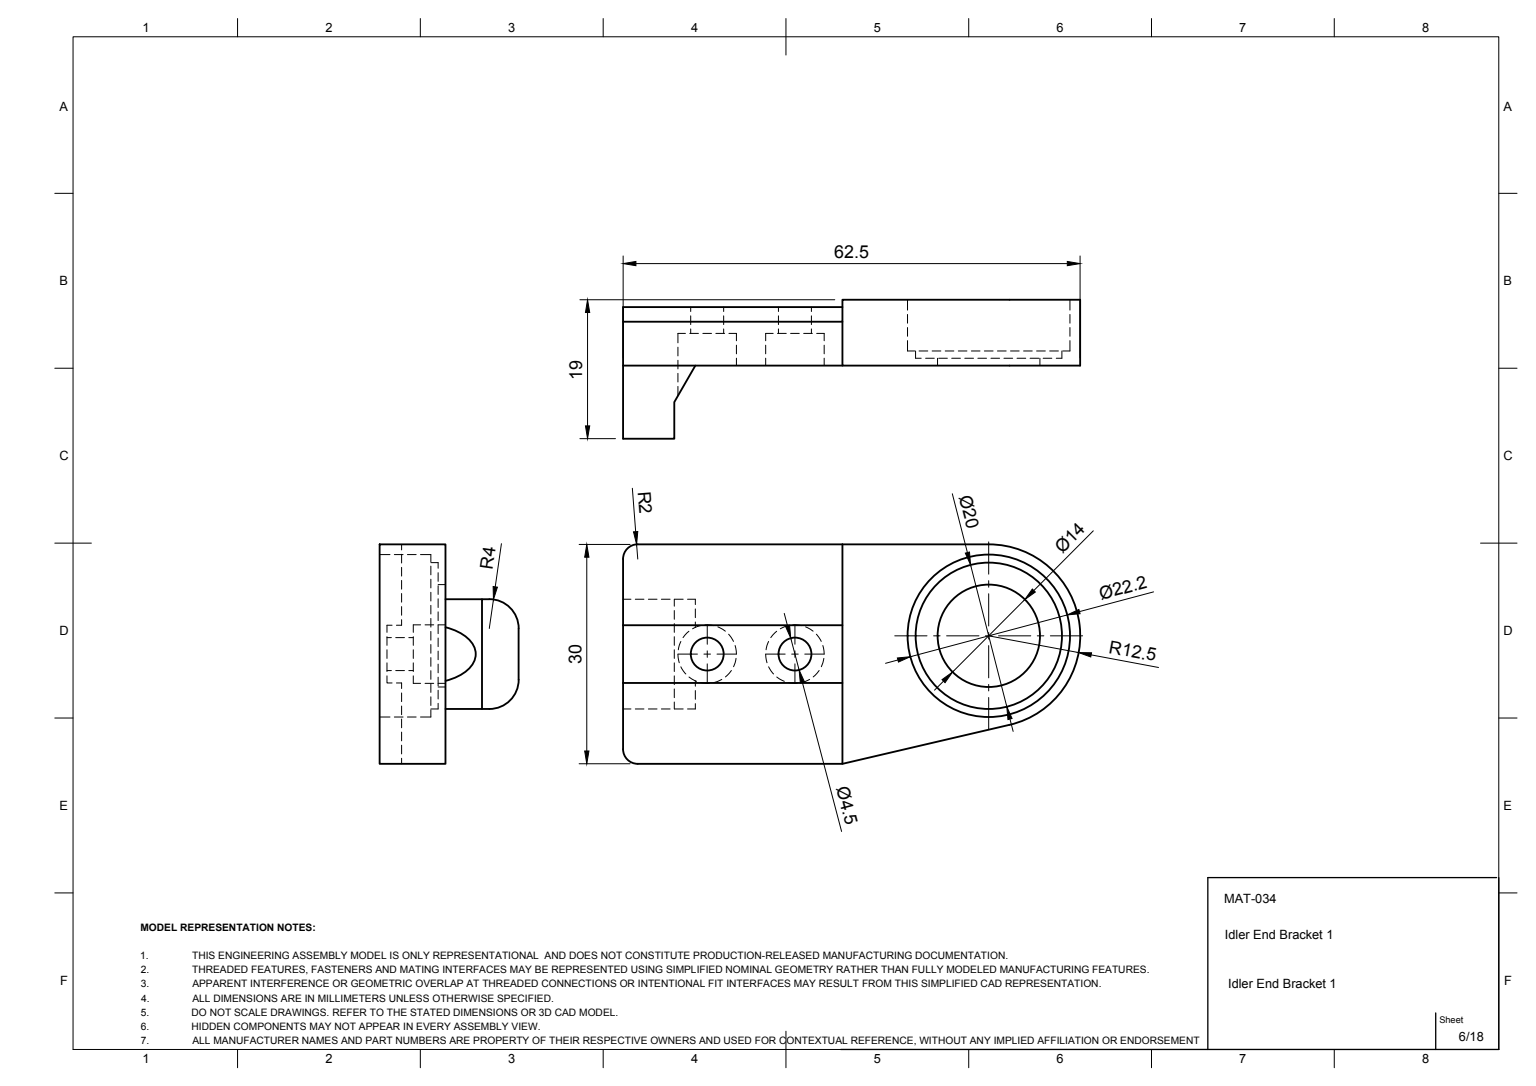
ISO-10303-21;
HEADER;
/* Generated by software containing ST-Developer
 * from STEP Tools, Inc. (www.steptools.com) 
 */

FILE_DESCRIPTION(
/* description */ ('STEP AP214'),
/* implementation_level */ '2;1');

FILE_NAME(
/* name */ 'Idler End Bracket 1.step',
/* time_stamp */ '2026-11-14T09:24:36-08:00',
/* author */ (''),
/* organization */ (''),
/* preprocessor_version */ 'ST-DEVELOPER v20.2',
/* originating_system */ 'Autodesk Translation Framework v15.17.0.0',
/* authorisation */ '');

FILE_SCHEMA (('AUTOMOTIVE_DESIGN { 1 0 10303 214 3 1 1 }'));
ENDSEC;

DATA;
#10=MECHANICAL_DESIGN_GEOMETRIC_PRESENTATION_REPRESENTATION('',(#205),#18867);
#167=ELLIPSE('',#11309,7.99999999999913,3.99999999999963);
#168=ELLIPSE('',#11311,7.99999999999913,3.99999999999963);
#173=SHAPE_REPRESENTATION_RELATIONSHIP('SRR','None',#18937,#189);
#189=ADVANCED_BREP_SHAPE_REPRESENTATION('',(#229),#18853);
#205=STYLED_ITEM('',(#19024),#229);
#229=MANIFOLD_SOLID_BREP('Body1',#10960);
#283=FACE_BOUND('',#1465,.T.);
#284=FACE_BOUND('',#1466,.T.);
#285=FACE_BOUND('',#1468,.T.);
#286=FACE_BOUND('',#1470,.T.);
#287=FACE_BOUND('',#1472,.T.);
#288=FACE_BOUND('',#1476,.T.);
#289=FACE_BOUND('',#1478,.T.);
#290=FACE_BOUND('',#1487,.T.);
#291=FACE_BOUND('',#1488,.T.);
#453=PLANE('',#11330);
#454=PLANE('',#11332);
#455=PLANE('',#11334);
#456=PLANE('',#11335);
#457=PLANE('',#11339);
#458=PLANE('',#11340);
#459=PLANE('',#11343);
#460=PLANE('',#11344);
#461=PLANE('',#11347);
#462=PLANE('',#11348);
#463=PLANE('',#11349);
#464=PLANE('',#11352);
#465=PLANE('',#11353);
#466=PLANE('',#11354);
#467=PLANE('',#11355);
#468=PLANE('',#11358);
#469=PLANE('',#11359);
#470=PLANE('',#11362);
#471=PLANE('',#11363);
#472=PLANE('',#11364);
#473=PLANE('',#11365);
#821=FACE_OUTER_BOUND('',#1449,.T.);
#822=FACE_OUTER_BOUND('',#1450,.T.);
#823=FACE_OUTER_BOUND('',#1451,.T.);
#824=FACE_OUTER_BOUND('',#1452,.T.);
#825=FACE_OUTER_BOUND('',#1453,.T.);
#826=FACE_OUTER_BOUND('',#1454,.T.);
#827=FACE_OUTER_BOUND('',#1455,.T.);
#828=FACE_OUTER_BOUND('',#1456,.T.);
#829=FACE_OUTER_BOUND('',#1457,.T.);
#830=FACE_OUTER_BOUND('',#1458,.T.);
#831=FACE_OUTER_BOUND('',#1459,.T.);
#832=FACE_OUTER_BOUND('',#1460,.T.);
#833=FACE_OUTER_BOUND('',#1461,.T.);
#834=FACE_OUTER_BOUND('',#1462,.T.);
#835=FACE_OUTER_BOUND('',#1463,.T.);
#836=FACE_OUTER_BOUND('',#1464,.T.);
#837=FACE_OUTER_BOUND('',#1467,.T.);
#838=FACE_OUTER_BOUND('',#1469,.T.);
#839=FACE_OUTER_BOUND('',#1471,.T.);
#840=FACE_OUTER_BOUND('',#1473,.T.);
#841=FACE_OUTER_BOUND('',#1474,.T.);
#842=FACE_OUTER_BOUND('',#1475,.T.);
#843=FACE_OUTER_BOUND('',#1477,.T.);
#844=FACE_OUTER_BOUND('',#1479,.T.);
#845=FACE_OUTER_BOUND('',#1480,.T.);
#846=FACE_OUTER_BOUND('',#1481,.T.);
#847=FACE_OUTER_BOUND('',#1482,.T.);
#848=FACE_OUTER_BOUND('',#1483,.T.);
#849=FACE_OUTER_BOUND('',#1484,.T.);
#850=FACE_OUTER_BOUND('',#1485,.T.);
#851=FACE_OUTER_BOUND('',#1486,.T.);
#852=FACE_OUTER_BOUND('',#1489,.T.);
#853=FACE_OUTER_BOUND('',#1490,.T.);
#1449=EDGE_LOOP('',(#7584,#7585,#7586,#7587,#7588,#7589));
#1450=EDGE_LOOP('',(#7590,#7591,#7592,#7593));
#1451=EDGE_LOOP('',(#7594,#7595,#7596,#7597));
#1452=EDGE_LOOP('',(#7598,#7599,#7600,#7601));
#1453=EDGE_LOOP('',(#7602,#7603,#7604,#7605));
#1454=EDGE_LOOP('',(#7606,#7607,#7608,#7609));
#1455=EDGE_LOOP('',(#7610,#7611,#7612,#7613));
#1456=EDGE_LOOP('',(#7614,#7615,#7616,#7617,#7618));
#1457=EDGE_LOOP('',(#7619,#7620,#7621,#7622,#7623));
#1458=EDGE_LOOP('',(#7624,#7625,#7626,#7627,#7628,#7629,#7630,#7631));
#1459=EDGE_LOOP('',(#7632,#7633,#7634,#7635,#7636));
#1460=EDGE_LOOP('',(#7637,#7638,#7639,#7640));
#1461=EDGE_LOOP('',(#7641,#7642,#7643,#7644,#7645,#7646));
#1462=EDGE_LOOP('',(#7647,#7648,#7649,#7650,#7651,#7652,#7653,#7654,#7655,
#7656,#7657,#7658,#7659,#7660));
#1463=EDGE_LOOP('',(#7661,#7662,#7663,#7664));
#1464=EDGE_LOOP('',(#7665,#7666,#7667,#7668,#7669,#7670,#7671,#7672,#7673,
#7674,#7675,#7676,#7677));
#1465=EDGE_LOOP('',(#7678));
#1466=EDGE_LOOP('',(#7679));
#1467=EDGE_LOOP('',(#7680,#7681,#7682,#7683));
#1468=EDGE_LOOP('',(#7684));
#1469=EDGE_LOOP('',(#7685));
#1470=EDGE_LOOP('',(#7686));
#1471=EDGE_LOOP('',(#7687));
#1472=EDGE_LOOP('',(#7688));
#1473=EDGE_LOOP('',(#7689,#7690,#7691,#7692));
#1474=EDGE_LOOP('',(#7693,#7694,#7695,#7696));
#1475=EDGE_LOOP('',(#7697));
#1476=EDGE_LOOP('',(#7698));
#1477=EDGE_LOOP('',(#7699));
#1478=EDGE_LOOP('',(#7700));
#1479=EDGE_LOOP('',(#7701,#7702,#7703,#7704,#7705));
#1480=EDGE_LOOP('',(#7706,#7707,#7708,#7709,#7710,#7711));
#1481=EDGE_LOOP('',(#7712,#7713,#7714,#7715,#7716));
#1482=EDGE_LOOP('',(#7717,#7718,#7719,#7720));
#1483=EDGE_LOOP('',(#7721,#7722,#7723,#7724));
#1484=EDGE_LOOP('',(#7725,#7726,#7727,#7728));
#1485=EDGE_LOOP('',(#7729,#7730,#7731,#7732,#7733,#7734,#7735));
#1486=EDGE_LOOP('',(#7736,#7737,#7738,#7739));
#1487=EDGE_LOOP('',(#7740));
#1488=EDGE_LOOP('',(#7741));
#1489=EDGE_LOOP('',(#7742,#7743,#7744,#7745));
#1490=EDGE_LOOP('',(#7746,#7747,#7748,#7749));
#2237=LINE('',#16105,#3251);
#2238=LINE('',#16115,#3252);
#2239=LINE('',#16121,#3253);
#2240=LINE('',#16127,#3254);
#2241=LINE('',#16133,#3255);
#2242=LINE('',#16139,#3256);
#2243=LINE('',#16145,#3257);
#2244=LINE('',#16150,#3258);
#2245=LINE('',#16152,#3259);
#2246=LINE('',#16154,#3260);
#2247=LINE('',#16157,#3261);
#2248=LINE('',#16161,#3262);
#2249=LINE('',#16163,#3263);
#2250=LINE('',#16167,#3264);
#2251=LINE('',#16168,#3265);
#2252=LINE('',#16171,#3266);
#2253=LINE('',#16173,#3267);
#2254=LINE('',#16174,#3268);
#2255=LINE('',#16176,#3269);
#2256=LINE('',#16178,#3270);
#2257=LINE('',#16179,#3271);
#2258=LINE('',#16182,#3272);
#2259=LINE('',#16184,#3273);
#2260=LINE('',#16186,#3274);
#2261=LINE('',#16187,#3275);
#2262=LINE('',#16193,#3276);
#2263=LINE('',#16195,#3277);
#2264=LINE('',#16197,#3278);
#2265=LINE('',#16198,#3279);
#2266=LINE('',#16201,#3280);
#2267=LINE('',#16203,#3281);
#2268=LINE('',#16205,#3282);
#2269=LINE('',#16209,#3283);
#2270=LINE('',#16213,#3284);
#2271=LINE('',#16215,#3285);
#2272=LINE('',#16216,#3286);
#2273=LINE('',#16218,#3287);
#2274=LINE('',#16220,#3288);
#2275=LINE('',#16221,#3289);
#2276=LINE('',#16224,#3290);
#2277=LINE('',#16225,#3291);
#2278=LINE('',#16228,#3292);
#2279=LINE('',#16232,#3293);
#2280=LINE('',#16233,#3294);
#2281=LINE('',#16234,#3295);
#2282=LINE('',#16245,#3296);
#2283=LINE('',#16246,#3297);
#2284=LINE('',#16247,#3298);
#2285=LINE('',#16252,#3299);
#2286=LINE('',#16256,#3300);
#2287=LINE('',#16257,#3301);
#2288=LINE('',#16259,#3302);
#2289=LINE('',#16260,#3303);
#2290=LINE('',#16262,#3304);
#2291=LINE('',#16263,#3305);
#2292=LINE('',#16268,#3306);
#2293=LINE('',#16269,#3307);
#3251=VECTOR('',#12793,4.);
#3252=VECTOR('',#12804,2.25);
#3253=VECTOR('',#12811,4.);
#3254=VECTOR('',#12818,2.25);
#3255=VECTOR('',#12825,7.00000000000001);
#3256=VECTOR('',#12832,10.);
#3257=VECTOR('',#12839,11.1);
#3258=VECTOR('',#12844,1000.);
#3259=VECTOR('',#12845,1000.);
#3260=VECTOR('',#12846,1000.);
#3261=VECTOR('',#12849,1000.);
#3262=VECTOR('',#12852,1000.);
#3263=VECTOR('',#12853,1000.);
#3264=VECTOR('',#12856,1000.);
#3265=VECTOR('',#12857,1000.);
#3266=VECTOR('',#12860,1000.);
#3267=VECTOR('',#12861,1000.);
#3268=VECTOR('',#12862,1000.);
#3269=VECTOR('',#12863,1000.);
#3270=VECTOR('',#12864,1000.);
#3271=VECTOR('',#12865,1000.);
#3272=VECTOR('',#12868,1000.);
#3273=VECTOR('',#12869,1000.);
#3274=VECTOR('',#12870,1000.);
#3275=VECTOR('',#12871,1000.);
#3276=VECTOR('',#12878,1000.);
#3277=VECTOR('',#12881,1000.);
#3278=VECTOR('',#12882,1000.);
#3279=VECTOR('',#12883,1000.);
#3280=VECTOR('',#12886,1000.);
#3281=VECTOR('',#12887,1000.);
#3282=VECTOR('',#12888,1000.);
#3283=VECTOR('',#12891,1000.);
#3284=VECTOR('',#12894,1000.);
#3285=VECTOR('',#12895,1000.);
#3286=VECTOR('',#12896,1000.);
#3287=VECTOR('',#12897,1000.);
#3288=VECTOR('',#12898,1000.);
#3289=VECTOR('',#12899,1000.);
#3290=VECTOR('',#12902,1000.);
#3291=VECTOR('',#12903,1000.);
#3292=VECTOR('',#12906,1000.);
#3293=VECTOR('',#12911,1000.);
#3294=VECTOR('',#12912,1000.);
#3295=VECTOR('',#12913,1000.);
#3296=VECTOR('',#12930,1000.);
#3297=VECTOR('',#12931,1000.);
#3298=VECTOR('',#12932,1000.);
#3299=VECTOR('',#12937,1000.);
#3300=VECTOR('',#12940,1000.);
#3301=VECTOR('',#12941,1000.);
#3302=VECTOR('',#12944,1000.);
#3303=VECTOR('',#12945,1000.);
#3304=VECTOR('',#12948,1000.);
#3305=VECTOR('',#12949,1000.);
#3306=VECTOR('',#12958,1000.);
#3307=VECTOR('',#12959,1000.);
#4123=CIRCLE('',#11308,4.);
#4124=CIRCLE('',#11310,4.);
#4125=CIRCLE('',#11313,2.25);
#4126=CIRCLE('',#11314,2.25);
#4127=CIRCLE('',#11316,4.);
#4128=CIRCLE('',#11317,4.);
#4129=CIRCLE('',#11319,2.25);
#4130=CIRCLE('',#11320,2.25);
#4131=CIRCLE('',#11322,7.00000000000001);
#4132=CIRCLE('',#11323,7.00000000000001);
#4133=CIRCLE('',#11325,10.);
#4134=CIRCLE('',#11326,10.);
#4135=CIRCLE('',#11328,11.1);
#4136=CIRCLE('',#11329,11.1);
#4137=CIRCLE('',#11331,2.);
#4138=CIRCLE('',#11333,2.);
#4139=CIRCLE('',#11337,12.5);
#4140=CIRCLE('',#11338,12.5);
#4141=CIRCLE('',#11341,4.);
#4142=CIRCLE('',#11342,4.);
#4143=CIRCLE('',#11345,2.);
#4144=CIRCLE('',#11346,2.);
#4145=CIRCLE('',#11356,4.);
#4146=CIRCLE('',#11357,4.);
#4732=VERTEX_POINT('',#16102);
#4733=VERTEX_POINT('',#16104);
#4734=VERTEX_POINT('',#16106);
#4735=VERTEX_POINT('',#16108);
#4736=VERTEX_POINT('',#16112);
#4737=VERTEX_POINT('',#16114);
#4738=VERTEX_POINT('',#16118);
#4739=VERTEX_POINT('',#16120);
#4740=VERTEX_POINT('',#16124);
#4741=VERTEX_POINT('',#16126);
#4742=VERTEX_POINT('',#16130);
#4743=VERTEX_POINT('',#16132);
#4744=VERTEX_POINT('',#16136);
#4745=VERTEX_POINT('',#16138);
#4746=VERTEX_POINT('',#16142);
#4747=VERTEX_POINT('',#16144);
#4748=VERTEX_POINT('',#16148);
#4749=VERTEX_POINT('',#16149);
#4750=VERTEX_POINT('',#16151);
#4751=VERTEX_POINT('',#16153);
#4752=VERTEX_POINT('',#16155);
#4753=VERTEX_POINT('',#16159);
#4754=VERTEX_POINT('',#16160);
#4755=VERTEX_POINT('',#16162);
#4756=VERTEX_POINT('',#16164);
#4757=VERTEX_POINT('',#16166);
#4758=VERTEX_POINT('',#16170);
#4759=VERTEX_POINT('',#16172);
#4760=VERTEX_POINT('',#16175);
#4761=VERTEX_POINT('',#16177);
#4762=VERTEX_POINT('',#16181);
#4763=VERTEX_POINT('',#16183);
#4764=VERTEX_POINT('',#16185);
#4765=VERTEX_POINT('',#16189);
#4766=VERTEX_POINT('',#16191);
#4767=VERTEX_POINT('',#16196);
#4768=VERTEX_POINT('',#16200);
#4769=VERTEX_POINT('',#16202);
#4770=VERTEX_POINT('',#16204);
#4771=VERTEX_POINT('',#16206);
#4772=VERTEX_POINT('',#16208);
#4773=VERTEX_POINT('',#16210);
#4774=VERTEX_POINT('',#16212);
#4775=VERTEX_POINT('',#16214);
#4776=VERTEX_POINT('',#16217);
#4777=VERTEX_POINT('',#16219);
#4778=VERTEX_POINT('',#16223);
#4779=VERTEX_POINT('',#16227);
#4780=VERTEX_POINT('',#16231);
#4781=VERTEX_POINT('',#16243);
#4782=VERTEX_POINT('',#16244);
#4783=VERTEX_POINT('',#16249);
#4784=VERTEX_POINT('',#16251);
#4785=VERTEX_POINT('',#16253);
#4786=VERTEX_POINT('',#16255);
#5825=EDGE_CURVE('',#4732,#4732,#4123,.T.);
#5826=EDGE_CURVE('',#4732,#4733,#2237,.T.);
#5827=EDGE_CURVE('',#4734,#4733,#167,.T.);
#5828=EDGE_CURVE('',#4735,#4734,#4124,.T.);
#5829=EDGE_CURVE('',#4733,#4735,#168,.T.);
#5830=EDGE_CURVE('',#4736,#4736,#4125,.T.);
#5831=EDGE_CURVE('',#4736,#4737,#2238,.T.);
#5832=EDGE_CURVE('',#4737,#4737,#4126,.T.);
#5833=EDGE_CURVE('',#4738,#4738,#4127,.T.);
#5834=EDGE_CURVE('',#4738,#4739,#2239,.T.);
#5835=EDGE_CURVE('',#4739,#4739,#4128,.T.);
#5836=EDGE_CURVE('',#4740,#4740,#4129,.T.);
#5837=EDGE_CURVE('',#4740,#4741,#2240,.T.);
#5838=EDGE_CURVE('',#4741,#4741,#4130,.T.);
#5839=EDGE_CURVE('',#4742,#4742,#4131,.T.);
#5840=EDGE_CURVE('',#4742,#4743,#2241,.T.);
#5841=EDGE_CURVE('',#4743,#4743,#4132,.T.);
#5842=EDGE_CURVE('',#4744,#4744,#4133,.T.);
#5843=EDGE_CURVE('',#4744,#4745,#2242,.T.);
#5844=EDGE_CURVE('',#4745,#4745,#4134,.T.);
#5845=EDGE_CURVE('',#4746,#4746,#4135,.T.);
#5846=EDGE_CURVE('',#4746,#4747,#2243,.T.);
#5847=EDGE_CURVE('',#4747,#4747,#4136,.T.);
#5848=EDGE_CURVE('',#4748,#4749,#2244,.T.);
#5849=EDGE_CURVE('',#4749,#4750,#2245,.T.);
#5850=EDGE_CURVE('',#4751,#4750,#2246,.T.);
#5851=EDGE_CURVE('',#4752,#4751,#4137,.T.);
#5852=EDGE_CURVE('',#4748,#4752,#2247,.T.);
#5853=EDGE_CURVE('',#4753,#4754,#2248,.T.);
#5854=EDGE_CURVE('',#4755,#4754,#2249,.T.);
#5855=EDGE_CURVE('',#4756,#4755,#4138,.T.);
#5856=EDGE_CURVE('',#4756,#4757,#2250,.T.);
#5857=EDGE_CURVE('',#4757,#4753,#2251,.T.);
#5858=EDGE_CURVE('',#4758,#4749,#2252,.T.);
#5859=EDGE_CURVE('',#4758,#4759,#2253,.T.);
#5860=EDGE_CURVE('',#4759,#4753,#2254,.T.);
#5861=EDGE_CURVE('',#4757,#4760,#2255,.T.);
#5862=EDGE_CURVE('',#4760,#4761,#2256,.T.);
#5863=EDGE_CURVE('',#4750,#4761,#2257,.T.);
#5864=EDGE_CURVE('',#4762,#4760,#2258,.T.);
#5865=EDGE_CURVE('',#4763,#4757,#2259,.T.);
#5866=EDGE_CURVE('',#4764,#4763,#2260,.T.);
#5867=EDGE_CURVE('',#4764,#4762,#2261,.T.);
#5868=EDGE_CURVE('',#4762,#4765,#4139,.T.);
#5869=EDGE_CURVE('',#4764,#4766,#4140,.T.);
#5870=EDGE_CURVE('',#4766,#4765,#2262,.T.);
#5871=EDGE_CURVE('',#4761,#4765,#2263,.T.);
#5872=EDGE_CURVE('',#4767,#4766,#2264,.T.);
#5873=EDGE_CURVE('',#4751,#4767,#2265,.T.);
#5874=EDGE_CURVE('',#4768,#4752,#2266,.T.);
#5875=EDGE_CURVE('',#4768,#4769,#2267,.T.);
#5876=EDGE_CURVE('',#4770,#4769,#2268,.T.);
#5877=EDGE_CURVE('',#4771,#4770,#4141,.T.);
#5878=EDGE_CURVE('',#4771,#4772,#2269,.T.);
#5879=EDGE_CURVE('',#4773,#4772,#4142,.T.);
#5880=EDGE_CURVE('',#4773,#4774,#2270,.T.);
#5881=EDGE_CURVE('',#4774,#4775,#2271,.T.);
#5882=EDGE_CURVE('',#4755,#4775,#2272,.T.);
#5883=EDGE_CURVE('',#4776,#4754,#2273,.T.);
#5884=EDGE_CURVE('',#4776,#4777,#2274,.T.);
#5885=EDGE_CURVE('',#4777,#4748,#2275,.T.);
#5886=EDGE_CURVE('',#4778,#4756,#2276,.T.);
#5887=EDGE_CURVE('',#4778,#4763,#2277,.T.);
#5888=EDGE_CURVE('',#4779,#4769,#2278,.T.);
#5889=EDGE_CURVE('',#4767,#4768,#4143,.T.);
#5890=EDGE_CURVE('',#4775,#4778,#4144,.T.);
#5891=EDGE_CURVE('',#4774,#4780,#2279,.T.);
#5892=EDGE_CURVE('',#4735,#4780,#2280,.T.);
#5893=EDGE_CURVE('',#4779,#4734,#2281,.T.);
#5894=EDGE_CURVE('',#4781,#4782,#2282,.T.);
#5895=EDGE_CURVE('',#4780,#4782,#2283,.T.);
#5896=EDGE_CURVE('',#4781,#4773,#2284,.T.);
#5897=EDGE_CURVE('',#4783,#4781,#4145,.T.);
#5898=EDGE_CURVE('',#4783,#4784,#2285,.T.);
#5899=EDGE_CURVE('',#4785,#4784,#4146,.T.);
#5900=EDGE_CURVE('',#4785,#4786,#2286,.T.);
#5901=EDGE_CURVE('',#4782,#4786,#2287,.T.);
#5902=EDGE_CURVE('',#4786,#4779,#2288,.T.);
#5903=EDGE_CURVE('',#4770,#4785,#2289,.T.);
#5904=EDGE_CURVE('',#4772,#4783,#2290,.T.);
#5905=EDGE_CURVE('',#4784,#4771,#2291,.T.);
#5906=EDGE_CURVE('',#4759,#4776,#2292,.T.);
#5907=EDGE_CURVE('',#4777,#4758,#2293,.T.);
#7584=ORIENTED_EDGE('',*,*,#5825,.T.);
#7585=ORIENTED_EDGE('',*,*,#5826,.T.);
#7586=ORIENTED_EDGE('',*,*,#5827,.F.);
#7587=ORIENTED_EDGE('',*,*,#5828,.F.);
#7588=ORIENTED_EDGE('',*,*,#5829,.F.);
#7589=ORIENTED_EDGE('',*,*,#5826,.F.);
#7590=ORIENTED_EDGE('',*,*,#5830,.F.);
#7591=ORIENTED_EDGE('',*,*,#5831,.T.);
#7592=ORIENTED_EDGE('',*,*,#5832,.F.);
#7593=ORIENTED_EDGE('',*,*,#5831,.F.);
#7594=ORIENTED_EDGE('',*,*,#5833,.T.);
#7595=ORIENTED_EDGE('',*,*,#5834,.T.);
#7596=ORIENTED_EDGE('',*,*,#5835,.F.);
#7597=ORIENTED_EDGE('',*,*,#5834,.F.);
#7598=ORIENTED_EDGE('',*,*,#5836,.F.);
#7599=ORIENTED_EDGE('',*,*,#5837,.T.);
#7600=ORIENTED_EDGE('',*,*,#5838,.F.);
#7601=ORIENTED_EDGE('',*,*,#5837,.F.);
#7602=ORIENTED_EDGE('',*,*,#5839,.T.);
#7603=ORIENTED_EDGE('',*,*,#5840,.T.);
#7604=ORIENTED_EDGE('',*,*,#5841,.F.);
#7605=ORIENTED_EDGE('',*,*,#5840,.F.);
#7606=ORIENTED_EDGE('',*,*,#5842,.T.);
#7607=ORIENTED_EDGE('',*,*,#5843,.T.);
#7608=ORIENTED_EDGE('',*,*,#5844,.F.);
#7609=ORIENTED_EDGE('',*,*,#5843,.F.);
#7610=ORIENTED_EDGE('',*,*,#5845,.T.);
#7611=ORIENTED_EDGE('',*,*,#5846,.T.);
#7612=ORIENTED_EDGE('',*,*,#5847,.F.);
#7613=ORIENTED_EDGE('',*,*,#5846,.F.);
#7614=ORIENTED_EDGE('',*,*,#5848,.T.);
#7615=ORIENTED_EDGE('',*,*,#5849,.T.);
#7616=ORIENTED_EDGE('',*,*,#5850,.F.);
#7617=ORIENTED_EDGE('',*,*,#5851,.F.);
#7618=ORIENTED_EDGE('',*,*,#5852,.F.);
#7619=ORIENTED_EDGE('',*,*,#5853,.T.);
#7620=ORIENTED_EDGE('',*,*,#5854,.F.);
#7621=ORIENTED_EDGE('',*,*,#5855,.F.);
#7622=ORIENTED_EDGE('',*,*,#5856,.T.);
#7623=ORIENTED_EDGE('',*,*,#5857,.T.);
#7624=ORIENTED_EDGE('',*,*,#5858,.F.);
#7625=ORIENTED_EDGE('',*,*,#5859,.T.);
#7626=ORIENTED_EDGE('',*,*,#5860,.T.);
#7627=ORIENTED_EDGE('',*,*,#5857,.F.);
#7628=ORIENTED_EDGE('',*,*,#5861,.T.);
#7629=ORIENTED_EDGE('',*,*,#5862,.T.);
#7630=ORIENTED_EDGE('',*,*,#5863,.F.);
#7631=ORIENTED_EDGE('',*,*,#5849,.F.);
#7632=ORIENTED_EDGE('',*,*,#5864,.T.);
#7633=ORIENTED_EDGE('',*,*,#5861,.F.);
#7634=ORIENTED_EDGE('',*,*,#5865,.F.);
#7635=ORIENTED_EDGE('',*,*,#5866,.F.);
#7636=ORIENTED_EDGE('',*,*,#5867,.T.);
#7637=ORIENTED_EDGE('',*,*,#5868,.F.);
#7638=ORIENTED_EDGE('',*,*,#5867,.F.);
#7639=ORIENTED_EDGE('',*,*,#5869,.T.);
#7640=ORIENTED_EDGE('',*,*,#5870,.T.);
#7641=ORIENTED_EDGE('',*,*,#5863,.T.);
#7642=ORIENTED_EDGE('',*,*,#5871,.T.);
#7643=ORIENTED_EDGE('',*,*,#5870,.F.);
#7644=ORIENTED_EDGE('',*,*,#5872,.F.);
#7645=ORIENTED_EDGE('',*,*,#5873,.F.);
#7646=ORIENTED_EDGE('',*,*,#5850,.T.);
#7647=ORIENTED_EDGE('',*,*,#5874,.F.);
#7648=ORIENTED_EDGE('',*,*,#5875,.T.);
#7649=ORIENTED_EDGE('',*,*,#5876,.F.);
#7650=ORIENTED_EDGE('',*,*,#5877,.F.);
#7651=ORIENTED_EDGE('',*,*,#5878,.T.);
#7652=ORIENTED_EDGE('',*,*,#5879,.F.);
#7653=ORIENTED_EDGE('',*,*,#5880,.T.);
#7654=ORIENTED_EDGE('',*,*,#5881,.T.);
#7655=ORIENTED_EDGE('',*,*,#5882,.F.);
#7656=ORIENTED_EDGE('',*,*,#5854,.T.);
#7657=ORIENTED_EDGE('',*,*,#5883,.F.);
#7658=ORIENTED_EDGE('',*,*,#5884,.T.);
#7659=ORIENTED_EDGE('',*,*,#5885,.T.);
#7660=ORIENTED_EDGE('',*,*,#5852,.T.);
#7661=ORIENTED_EDGE('',*,*,#5886,.F.);
#7662=ORIENTED_EDGE('',*,*,#5887,.T.);
#7663=ORIENTED_EDGE('',*,*,#5865,.T.);
#7664=ORIENTED_EDGE('',*,*,#5856,.F.);
#7665=ORIENTED_EDGE('',*,*,#5888,.T.);
#7666=ORIENTED_EDGE('',*,*,#5875,.F.);
#7667=ORIENTED_EDGE('',*,*,#5889,.F.);
#7668=ORIENTED_EDGE('',*,*,#5872,.T.);
#7669=ORIENTED_EDGE('',*,*,#5869,.F.);
#7670=ORIENTED_EDGE('',*,*,#5866,.T.);
#7671=ORIENTED_EDGE('',*,*,#5887,.F.);
#7672=ORIENTED_EDGE('',*,*,#5890,.F.);
#7673=ORIENTED_EDGE('',*,*,#5881,.F.);
#7674=ORIENTED_EDGE('',*,*,#5891,.T.);
#7675=ORIENTED_EDGE('',*,*,#5892,.F.);
#7676=ORIENTED_EDGE('',*,*,#5828,.T.);
#7677=ORIENTED_EDGE('',*,*,#5893,.F.);
#7678=ORIENTED_EDGE('',*,*,#5835,.T.);
#7679=ORIENTED_EDGE('',*,*,#5839,.F.);
#7680=ORIENTED_EDGE('',*,*,#5864,.F.);
#7681=ORIENTED_EDGE('',*,*,#5868,.T.);
#7682=ORIENTED_EDGE('',*,*,#5871,.F.);
#7683=ORIENTED_EDGE('',*,*,#5862,.F.);
#7684=ORIENTED_EDGE('',*,*,#5847,.T.);
#7685=ORIENTED_EDGE('',*,*,#5845,.F.);
#7686=ORIENTED_EDGE('',*,*,#5844,.T.);
#7687=ORIENTED_EDGE('',*,*,#5842,.F.);
#7688=ORIENTED_EDGE('',*,*,#5841,.T.);
#7689=ORIENTED_EDGE('',*,*,#5855,.T.);
#7690=ORIENTED_EDGE('',*,*,#5882,.T.);
#7691=ORIENTED_EDGE('',*,*,#5890,.T.);
#7692=ORIENTED_EDGE('',*,*,#5886,.T.);
#7693=ORIENTED_EDGE('',*,*,#5851,.T.);
#7694=ORIENTED_EDGE('',*,*,#5873,.T.);
#7695=ORIENTED_EDGE('',*,*,#5889,.T.);
#7696=ORIENTED_EDGE('',*,*,#5874,.T.);
#7697=ORIENTED_EDGE('',*,*,#5833,.F.);
#7698=ORIENTED_EDGE('',*,*,#5838,.T.);
#7699=ORIENTED_EDGE('',*,*,#5825,.F.);
#7700=ORIENTED_EDGE('',*,*,#5832,.T.);
#7701=ORIENTED_EDGE('',*,*,#5894,.T.);
#7702=ORIENTED_EDGE('',*,*,#5895,.F.);
#7703=ORIENTED_EDGE('',*,*,#5891,.F.);
#7704=ORIENTED_EDGE('',*,*,#5880,.F.);
#7705=ORIENTED_EDGE('',*,*,#5896,.F.);
#7706=ORIENTED_EDGE('',*,*,#5894,.F.);
#7707=ORIENTED_EDGE('',*,*,#5897,.F.);
#7708=ORIENTED_EDGE('',*,*,#5898,.T.);
#7709=ORIENTED_EDGE('',*,*,#5899,.F.);
#7710=ORIENTED_EDGE('',*,*,#5900,.T.);
#7711=ORIENTED_EDGE('',*,*,#5901,.F.);
#7712=ORIENTED_EDGE('',*,*,#5876,.T.);
#7713=ORIENTED_EDGE('',*,*,#5888,.F.);
#7714=ORIENTED_EDGE('',*,*,#5902,.F.);
#7715=ORIENTED_EDGE('',*,*,#5900,.F.);
#7716=ORIENTED_EDGE('',*,*,#5903,.F.);
#7717=ORIENTED_EDGE('',*,*,#5898,.F.);
#7718=ORIENTED_EDGE('',*,*,#5904,.F.);
#7719=ORIENTED_EDGE('',*,*,#5878,.F.);
#7720=ORIENTED_EDGE('',*,*,#5905,.F.);
#7721=ORIENTED_EDGE('',*,*,#5899,.T.);
#7722=ORIENTED_EDGE('',*,*,#5905,.T.);
#7723=ORIENTED_EDGE('',*,*,#5877,.T.);
#7724=ORIENTED_EDGE('',*,*,#5903,.T.);
#7725=ORIENTED_EDGE('',*,*,#5879,.T.);
#7726=ORIENTED_EDGE('',*,*,#5904,.T.);
#7727=ORIENTED_EDGE('',*,*,#5897,.T.);
#7728=ORIENTED_EDGE('',*,*,#5896,.T.);
#7729=ORIENTED_EDGE('',*,*,#5827,.T.);
#7730=ORIENTED_EDGE('',*,*,#5829,.T.);
#7731=ORIENTED_EDGE('',*,*,#5892,.T.);
#7732=ORIENTED_EDGE('',*,*,#5895,.T.);
#7733=ORIENTED_EDGE('',*,*,#5901,.T.);
#7734=ORIENTED_EDGE('',*,*,#5902,.T.);
#7735=ORIENTED_EDGE('',*,*,#5893,.T.);
#7736=ORIENTED_EDGE('',*,*,#5884,.F.);
#7737=ORIENTED_EDGE('',*,*,#5906,.F.);
#7738=ORIENTED_EDGE('',*,*,#5859,.F.);
#7739=ORIENTED_EDGE('',*,*,#5907,.F.);
#7740=ORIENTED_EDGE('',*,*,#5830,.T.);
#7741=ORIENTED_EDGE('',*,*,#5836,.T.);
#7742=ORIENTED_EDGE('',*,*,#5848,.F.);
#7743=ORIENTED_EDGE('',*,*,#5885,.F.);
#7744=ORIENTED_EDGE('',*,*,#5907,.T.);
#7745=ORIENTED_EDGE('',*,*,#5858,.T.);
#7746=ORIENTED_EDGE('',*,*,#5853,.F.);
#7747=ORIENTED_EDGE('',*,*,#5860,.F.);
#7748=ORIENTED_EDGE('',*,*,#5906,.T.);
#7749=ORIENTED_EDGE('',*,*,#5883,.T.);
#10174=CYLINDRICAL_SURFACE('',#11307,4.);
#10175=CYLINDRICAL_SURFACE('',#11312,2.25);
#10176=CYLINDRICAL_SURFACE('',#11315,4.);
#10177=CYLINDRICAL_SURFACE('',#11318,2.25);
#10178=CYLINDRICAL_SURFACE('',#11321,7.00000000000001);
#10179=CYLINDRICAL_SURFACE('',#11324,10.);
#10180=CYLINDRICAL_SURFACE('',#11327,11.1);
#10181=CYLINDRICAL_SURFACE('',#11336,12.5);
#10182=CYLINDRICAL_SURFACE('',#11350,2.);
#10183=CYLINDRICAL_SURFACE('',#11351,2.);
#10184=CYLINDRICAL_SURFACE('',#11360,4.);
#10185=CYLINDRICAL_SURFACE('',#11361,4.);
#10458=ADVANCED_FACE('',(#821),#10174,.F.);
#10459=ADVANCED_FACE('',(#822),#10175,.F.);
#10460=ADVANCED_FACE('',(#823),#10176,.F.);
#10461=ADVANCED_FACE('',(#824),#10177,.F.);
#10462=ADVANCED_FACE('',(#825),#10178,.F.);
#10463=ADVANCED_FACE('',(#826),#10179,.F.);
#10464=ADVANCED_FACE('',(#827),#10180,.F.);
#10465=ADVANCED_FACE('',(#828),#453,.F.);
#10466=ADVANCED_FACE('',(#829),#454,.F.);
#10467=ADVANCED_FACE('',(#830),#455,.F.);
#10468=ADVANCED_FACE('',(#831),#456,.T.);
#10469=ADVANCED_FACE('',(#832),#10181,.T.);
#10470=ADVANCED_FACE('',(#833),#457,.T.);
#10471=ADVANCED_FACE('',(#834),#458,.F.);
#10472=ADVANCED_FACE('',(#835),#459,.F.);
#10473=ADVANCED_FACE('',(#836,#283,#284),#460,.T.);
#10474=ADVANCED_FACE('',(#837,#285),#461,.F.);
#10475=ADVANCED_FACE('',(#838,#286),#462,.T.);
#10476=ADVANCED_FACE('',(#839,#287),#463,.T.);
#10477=ADVANCED_FACE('',(#840),#10182,.T.);
#10478=ADVANCED_FACE('',(#841),#10183,.T.);
#10479=ADVANCED_FACE('',(#842,#288),#464,.F.);
#10480=ADVANCED_FACE('',(#843,#289),#465,.F.);
#10481=ADVANCED_FACE('',(#844),#466,.F.);
#10482=ADVANCED_FACE('',(#845),#467,.F.);
#10483=ADVANCED_FACE('',(#846),#468,.F.);
#10484=ADVANCED_FACE('',(#847),#469,.T.);
#10485=ADVANCED_FACE('',(#848),#10184,.T.);
#10486=ADVANCED_FACE('',(#849),#10185,.T.);
#10487=ADVANCED_FACE('',(#850),#470,.F.);
#10488=ADVANCED_FACE('',(#851,#290,#291),#471,.F.);
#10489=ADVANCED_FACE('',(#852),#472,.F.);
#10490=ADVANCED_FACE('',(#853),#473,.F.);
#10960=CLOSED_SHELL('',(#10458,#10459,#10460,#10461,#10462,#10463,#10464,
#10465,#10466,#10467,#10468,#10469,#10470,#10471,#10472,#10473,#10474,#10475,
#10476,#10477,#10478,#10479,#10480,#10481,#10482,#10483,#10484,#10485,#10486,
#10487,#10488,#10489,#10490));
#11306=AXIS2_PLACEMENT_3D('',#16100,#12787,#12788);
#11307=AXIS2_PLACEMENT_3D('',#16101,#12789,#12790);
#11308=AXIS2_PLACEMENT_3D('',#16103,#12791,#12792);
#11309=AXIS2_PLACEMENT_3D('',#16107,#12794,#12795);
#11310=AXIS2_PLACEMENT_3D('',#16109,#12796,#12797);
#11311=AXIS2_PLACEMENT_3D('',#16110,#12798,#12799);
#11312=AXIS2_PLACEMENT_3D('',#16111,#12800,#12801);
#11313=AXIS2_PLACEMENT_3D('',#16113,#12802,#12803);
#11314=AXIS2_PLACEMENT_3D('',#16116,#12805,#12806);
#11315=AXIS2_PLACEMENT_3D('',#16117,#12807,#12808);
#11316=AXIS2_PLACEMENT_3D('',#16119,#12809,#12810);
#11317=AXIS2_PLACEMENT_3D('',#16122,#12812,#12813);
#11318=AXIS2_PLACEMENT_3D('',#16123,#12814,#12815);
#11319=AXIS2_PLACEMENT_3D('',#16125,#12816,#12817);
#11320=AXIS2_PLACEMENT_3D('',#16128,#12819,#12820);
#11321=AXIS2_PLACEMENT_3D('',#16129,#12821,#12822);
#11322=AXIS2_PLACEMENT_3D('',#16131,#12823,#12824);
#11323=AXIS2_PLACEMENT_3D('',#16134,#12826,#12827);
#11324=AXIS2_PLACEMENT_3D('',#16135,#12828,#12829);
#11325=AXIS2_PLACEMENT_3D('',#16137,#12830,#12831);
#11326=AXIS2_PLACEMENT_3D('',#16140,#12833,#12834);
#11327=AXIS2_PLACEMENT_3D('',#16141,#12835,#12836);
#11328=AXIS2_PLACEMENT_3D('',#16143,#12837,#12838);
#11329=AXIS2_PLACEMENT_3D('',#16146,#12840,#12841);
#11330=AXIS2_PLACEMENT_3D('',#16147,#12842,#12843);
#11331=AXIS2_PLACEMENT_3D('',#16156,#12847,#12848);
#11332=AXIS2_PLACEMENT_3D('',#16158,#12850,#12851);
#11333=AXIS2_PLACEMENT_3D('',#16165,#12854,#12855);
#11334=AXIS2_PLACEMENT_3D('',#16169,#12858,#12859);
#11335=AXIS2_PLACEMENT_3D('',#16180,#12866,#12867);
#11336=AXIS2_PLACEMENT_3D('',#16188,#12872,#12873);
#11337=AXIS2_PLACEMENT_3D('',#16190,#12874,#12875);
#11338=AXIS2_PLACEMENT_3D('',#16192,#12876,#12877);
#11339=AXIS2_PLACEMENT_3D('',#16194,#12879,#12880);
#11340=AXIS2_PLACEMENT_3D('',#16199,#12884,#12885);
#11341=AXIS2_PLACEMENT_3D('',#16207,#12889,#12890);
#11342=AXIS2_PLACEMENT_3D('',#16211,#12892,#12893);
#11343=AXIS2_PLACEMENT_3D('',#16222,#12900,#12901);
#11344=AXIS2_PLACEMENT_3D('',#16226,#12904,#12905);
#11345=AXIS2_PLACEMENT_3D('',#16229,#12907,#12908);
#11346=AXIS2_PLACEMENT_3D('',#16230,#12909,#12910);
#11347=AXIS2_PLACEMENT_3D('',#16235,#12914,#12915);
#11348=AXIS2_PLACEMENT_3D('',#16236,#12916,#12917);
#11349=AXIS2_PLACEMENT_3D('',#16237,#12918,#12919);
#11350=AXIS2_PLACEMENT_3D('',#16238,#12920,#12921);
#11351=AXIS2_PLACEMENT_3D('',#16239,#12922,#12923);
#11352=AXIS2_PLACEMENT_3D('',#16240,#12924,#12925);
#11353=AXIS2_PLACEMENT_3D('',#16241,#12926,#12927);
#11354=AXIS2_PLACEMENT_3D('',#16242,#12928,#12929);
#11355=AXIS2_PLACEMENT_3D('',#16248,#12933,#12934);
#11356=AXIS2_PLACEMENT_3D('',#16250,#12935,#12936);
#11357=AXIS2_PLACEMENT_3D('',#16254,#12938,#12939);
#11358=AXIS2_PLACEMENT_3D('',#16258,#12942,#12943);
#11359=AXIS2_PLACEMENT_3D('',#16261,#12946,#12947);
#11360=AXIS2_PLACEMENT_3D('',#16264,#12950,#12951);
#11361=AXIS2_PLACEMENT_3D('',#16265,#12952,#12953);
#11362=AXIS2_PLACEMENT_3D('',#16266,#12954,#12955);
#11363=AXIS2_PLACEMENT_3D('',#16267,#12956,#12957);
#11364=AXIS2_PLACEMENT_3D('',#16270,#12960,#12961);
#11365=AXIS2_PLACEMENT_3D('',#16271,#12962,#12963);
#12787=DIRECTION('axis',(0.,0.,1.));
#12788=DIRECTION('refdir',(1.,0.,0.));
#12789=DIRECTION('center_axis',(0.,0.,-1.));
#12790=DIRECTION('ref_axis',(1.,0.,0.));
#12791=DIRECTION('center_axis',(0.,0.,1.));
#12792=DIRECTION('ref_axis',(1.,0.,0.));
#12793=DIRECTION('',(0.,0.,-1.));
#12794=DIRECTION('center_axis',(-0.866025403784435,4.41270772476077E-16,
0.500000000000006));
#12795=DIRECTION('ref_axis',(0.500000000000006,5.55042661661472E-14,0.866025403784435));
#12796=DIRECTION('center_axis',(0.,0.,1.));
#12797=DIRECTION('ref_axis',(1.,0.,0.));
#12798=DIRECTION('center_axis',(-0.866025403784435,4.41270772476077E-16,
0.500000000000006));
#12799=DIRECTION('ref_axis',(0.500000000000006,5.55042661661472E-14,0.866025403784435));
#12800=DIRECTION('center_axis',(0.,0.,-1.));
#12801=DIRECTION('ref_axis',(1.,0.,0.));
#12802=DIRECTION('center_axis',(0.,0.,-1.));
#12803=DIRECTION('ref_axis',(-1.,0.,0.));
#12804=DIRECTION('',(0.,0.,-1.));
#12805=DIRECTION('center_axis',(0.,0.,1.));
#12806=DIRECTION('ref_axis',(1.,0.,0.));
#12807=DIRECTION('center_axis',(0.,0.,-1.));
#12808=DIRECTION('ref_axis',(1.,0.,0.));
#12809=DIRECTION('center_axis',(0.,0.,1.));
#12810=DIRECTION('ref_axis',(1.,0.,0.));
#12811=DIRECTION('',(0.,0.,-1.));
#12812=DIRECTION('center_axis',(0.,0.,1.));
#12813=DIRECTION('ref_axis',(1.,0.,0.));
#12814=DIRECTION('center_axis',(0.,0.,-1.));
#12815=DIRECTION('ref_axis',(1.,0.,0.));
#12816=DIRECTION('center_axis',(0.,0.,-1.));
#12817=DIRECTION('ref_axis',(-1.,0.,0.));
#12818=DIRECTION('',(0.,0.,-1.));
#12819=DIRECTION('center_axis',(0.,0.,1.));
#12820=DIRECTION('ref_axis',(1.,0.,0.));
#12821=DIRECTION('center_axis',(0.,0.,1.));
#12822=DIRECTION('ref_axis',(-1.,0.,0.));
#12823=DIRECTION('center_axis',(0.,0.,-1.));
#12824=DIRECTION('ref_axis',(-1.,0.,0.));
#12825=DIRECTION('',(0.,0.,1.));
#12826=DIRECTION('center_axis',(0.,0.,-1.));
#12827=DIRECTION('ref_axis',(-1.,0.,0.));
#12828=DIRECTION('center_axis',(0.,0.,1.));
#12829=DIRECTION('ref_axis',(-1.,0.,0.));
#12830=DIRECTION('center_axis',(0.,0.,-1.));
#12831=DIRECTION('ref_axis',(-1.,0.,0.));
#12832=DIRECTION('',(0.,0.,1.));
#12833=DIRECTION('center_axis',(0.,0.,-1.));
#12834=DIRECTION('ref_axis',(-1.,0.,0.));
#12835=DIRECTION('center_axis',(0.,0.,1.));
#12836=DIRECTION('ref_axis',(-1.,0.,0.));
#12837=DIRECTION('center_axis',(0.,0.,-1.));
#12838=DIRECTION('ref_axis',(-1.,0.,0.));
#12839=DIRECTION('',(0.,0.,1.));
#12840=DIRECTION('center_axis',(0.,0.,-1.));
#12841=DIRECTION('ref_axis',(-1.,0.,0.));
#12842=DIRECTION('center_axis',(0.,0.,-1.));
#12843=DIRECTION('ref_axis',(1.,0.,0.));
#12844=DIRECTION('',(1.,0.,0.));
#12845=DIRECTION('',(0.,1.,0.));
#12846=DIRECTION('',(1.,0.,0.));
#12847=DIRECTION('center_axis',(0.,0.,-1.));
#12848=DIRECTION('ref_axis',(1.,0.,0.));
#12849=DIRECTION('',(0.,1.,0.));
#12850=DIRECTION('center_axis',(0.,0.,-1.));
#12851=DIRECTION('ref_axis',(1.,0.,0.));
#12852=DIRECTION('',(-1.,-2.89120579329468E-17,0.));
#12853=DIRECTION('',(0.,1.,0.));
#12854=DIRECTION('center_axis',(0.,0.,-1.));
#12855=DIRECTION('ref_axis',(1.,0.,0.));
#12856=DIRECTION('',(1.,0.,0.));
#12857=DIRECTION('',(0.,1.,0.));
#12858=DIRECTION('center_axis',(1.,0.,0.));
#12859=DIRECTION('ref_axis',(0.,0.,1.));
#12860=DIRECTION('',(0.,0.,-1.));
#12861=DIRECTION('',(0.,-1.,0.));
#12862=DIRECTION('',(0.,0.,-1.));
#12863=DIRECTION('',(0.,0.,1.));
#12864=DIRECTION('',(0.,1.,0.));
#12865=DIRECTION('',(0.,0.,1.));
#12866=DIRECTION('center_axis',(0.227131156084319,-0.973864178382079,0.));
#12867=DIRECTION('ref_axis',(0.973864178382079,0.227131156084319,0.));
#12868=DIRECTION('',(-0.973864178382078,-0.227131156084319,0.));
#12869=DIRECTION('',(0.,0.,1.));
#12870=DIRECTION('',(-0.973864178382078,-0.227131156084319,0.));
#12871=DIRECTION('',(0.,0.,1.));
#12872=DIRECTION('center_axis',(0.,0.,1.));
#12873=DIRECTION('ref_axis',(0.993444557683537,0.114314963189256,0.));
#12874=DIRECTION('center_axis',(0.,0.,1.));
#12875=DIRECTION('ref_axis',(1.,0.,0.));
#12876=DIRECTION('center_axis',(0.,0.,1.));
#12877=DIRECTION('ref_axis',(1.,0.,0.));
#12878=DIRECTION('',(0.,0.,1.));
#12879=DIRECTION('center_axis',(0.,1.,0.));
#12880=DIRECTION('ref_axis',(0.,0.,-1.));
#12881=DIRECTION('',(1.,0.,0.));
#12882=DIRECTION('',(1.,0.,0.));
#12883=DIRECTION('',(0.,0.,-1.));
#12884=DIRECTION('center_axis',(1.,0.,0.));
#12885=DIRECTION('ref_axis',(0.,0.,1.));
#12886=DIRECTION('',(0.,0.,1.));
#12887=DIRECTION('',(0.,-1.,0.));
#12888=DIRECTION('',(0.,0.,1.));
#12889=DIRECTION('center_axis',(1.,0.,0.));
#12890=DIRECTION('ref_axis',(0.,0.,1.));
#12891=DIRECTION('',(0.,-1.,0.));
#12892=DIRECTION('center_axis',(1.,0.,0.));
#12893=DIRECTION('ref_axis',(0.,0.,1.));
#12894=DIRECTION('',(0.,0.,1.));
#12895=DIRECTION('',(0.,-1.,0.));
#12896=DIRECTION('',(0.,0.,-1.));
#12897=DIRECTION('',(0.,0.,-1.));
#12898=DIRECTION('',(0.,1.,0.));
#12899=DIRECTION('',(0.,0.,-1.));
#12900=DIRECTION('center_axis',(-1.15648231731787E-16,1.,0.));
#12901=DIRECTION('ref_axis',(-1.,-1.15648231731787E-16,0.));
#12902=DIRECTION('',(0.,0.,1.));
#12903=DIRECTION('',(1.,1.15648231731787E-16,0.));
#12904=DIRECTION('center_axis',(0.,0.,-1.));
#12905=DIRECTION('ref_axis',(1.,0.,0.));
#12906=DIRECTION('',(-1.,-1.23908819712629E-16,0.));
#12907=DIRECTION('center_axis',(0.,0.,1.));
#12908=DIRECTION('ref_axis',(1.,0.,0.));
#12909=DIRECTION('center_axis',(0.,0.,1.));
#12910=DIRECTION('ref_axis',(1.,0.,0.));
#12911=DIRECTION('',(1.,1.23908819712629E-16,0.));
#12912=DIRECTION('',(0.,-1.,0.));
#12913=DIRECTION('',(0.,-1.,0.));
#12914=DIRECTION('center_axis',(0.,0.,-1.));
#12915=DIRECTION('ref_axis',(1.,0.,0.));
#12916=DIRECTION('center_axis',(0.,0.,1.));
#12917=DIRECTION('ref_axis',(-1.,0.,0.));
#12918=DIRECTION('center_axis',(0.,0.,1.));
#12919=DIRECTION('ref_axis',(-1.,0.,0.));
#12920=DIRECTION('center_axis',(0.,0.,1.));
#12921=DIRECTION('ref_axis',(-1.,0.,0.));
#12922=DIRECTION('center_axis',(0.,0.,-1.));
#12923=DIRECTION('ref_axis',(1.,0.,0.));
#12924=DIRECTION('center_axis',(0.,0.,1.));
#12925=DIRECTION('ref_axis',(-1.,0.,0.));
#12926=DIRECTION('center_axis',(0.,0.,1.));
#12927=DIRECTION('ref_axis',(-1.,0.,0.));
#12928=DIRECTION('center_axis',(-1.23908819712629E-16,1.,0.));
#12929=DIRECTION('ref_axis',(-1.,-1.23908819712629E-16,0.));
#12930=DIRECTION('',(0.,0.,1.));
#12931=DIRECTION('',(-0.500000000000005,-6.19544098563151E-17,-0.866025403784436));
#12932=DIRECTION('',(-1.,-1.23908819712629E-16,0.));
#12933=DIRECTION('center_axis',(-1.,0.,0.));
#12934=DIRECTION('ref_axis',(0.,0.,-1.));
#12935=DIRECTION('center_axis',(-1.,0.,0.));
#12936=DIRECTION('ref_axis',(0.,0.,-1.));
#12937=DIRECTION('',(0.,1.,0.));
#12938=DIRECTION('center_axis',(-1.,0.,0.));
#12939=DIRECTION('ref_axis',(0.,0.,-1.));
#12940=DIRECTION('',(0.,0.,1.));
#12941=DIRECTION('',(0.,1.,0.));
#12942=DIRECTION('center_axis',(1.23908819712629E-16,-1.,0.));
#12943=DIRECTION('ref_axis',(1.,1.23908819712629E-16,0.));
#12944=DIRECTION('',(0.500000000000005,6.19544098563151E-17,0.866025403784436));
#12945=DIRECTION('',(1.,1.23908819712629E-16,0.));
#12946=DIRECTION('center_axis',(0.,0.,-1.));
#12947=DIRECTION('ref_axis',(1.,0.,0.));
#12948=DIRECTION('',(1.,1.23908819712629E-16,0.));
#12949=DIRECTION('',(-1.,-1.23908819712629E-16,0.));
#12950=DIRECTION('center_axis',(1.,1.23908819712629E-16,0.));
#12951=DIRECTION('ref_axis',(-1.23908819712629E-16,1.,0.));
#12952=DIRECTION('center_axis',(-1.,-1.23908819712629E-16,0.));
#12953=DIRECTION('ref_axis',(1.23908819712629E-16,-1.,0.));
#12954=DIRECTION('center_axis',(-0.866025403784436,0.,0.500000000000005));
#12955=DIRECTION('ref_axis',(0.,1.,0.));
#12956=DIRECTION('center_axis',(0.,0.,-1.));
#12957=DIRECTION('ref_axis',(1.,0.,0.));
#12958=DIRECTION('',(-1.,-2.89120579329468E-17,0.));
#12959=DIRECTION('',(1.,0.,0.));
#12960=DIRECTION('center_axis',(0.,-1.,0.));
#12961=DIRECTION('ref_axis',(0.,0.,1.));
#12962=DIRECTION('center_axis',(-2.89120579329468E-17,1.,0.));
#12963=DIRECTION('ref_axis',(-1.,-2.89120579329468E-17,0.));
#16100=CARTESIAN_POINT('',(0.,0.,0.));
#16101=CARTESIAN_POINT('Origin',(171.5,0.,-9.));
#16102=CARTESIAN_POINT('',(167.5,4.89858719658942E-16,-4.6));
#16103=CARTESIAN_POINT('Origin',(171.5,0.,-4.6));
#16104=CARTESIAN_POINT('',(167.5,4.89858719658966E-16,-13.1339745962156));
#16105=CARTESIAN_POINT('',(167.5,4.89858719658942E-16,-9.));
#16106=CARTESIAN_POINT('',(169.886751345948,3.66024982483438,-9.));
#16107=CARTESIAN_POINT('Origin',(171.5,3.67483821150927E-13,-6.20577136594092));
#16108=CARTESIAN_POINT('',(169.886751345948,-3.66024982483438,-9.));
#16109=CARTESIAN_POINT('Origin',(171.5,0.,-9.));
#16110=CARTESIAN_POINT('Origin',(171.5,3.67483821150927E-13,-6.20577136594092));
#16111=CARTESIAN_POINT('Origin',(171.5,0.,-9.));
#16112=CARTESIAN_POINT('',(169.25,2.75545529808155E-16,-1.));
#16113=CARTESIAN_POINT('Origin',(171.5,0.,-1.));
#16114=CARTESIAN_POINT('',(169.25,2.75545529808155E-16,-4.6));
#16115=CARTESIAN_POINT('',(169.25,2.75545529808155E-16,-9.));
#16116=CARTESIAN_POINT('Origin',(171.5,0.,-4.6));
#16117=CARTESIAN_POINT('Origin',(183.5,0.,-9.));
#16118=CARTESIAN_POINT('',(179.5,4.89858719658942E-16,-4.6));
#16119=CARTESIAN_POINT('Origin',(183.5,0.,-4.6));
#16120=CARTESIAN_POINT('',(179.5,4.89858719658942E-16,-9.));
#16121=CARTESIAN_POINT('',(179.5,4.89858719658942E-16,-9.));
#16122=CARTESIAN_POINT('Origin',(183.5,0.,-9.));
#16123=CARTESIAN_POINT('Origin',(183.5,0.,-9.));
#16124=CARTESIAN_POINT('',(181.25,2.75545529808155E-16,-1.));
#16125=CARTESIAN_POINT('Origin',(183.5,0.,-1.));
#16126=CARTESIAN_POINT('',(181.25,2.75545529808155E-16,-4.6));
#16127=CARTESIAN_POINT('',(181.25,2.75545529808155E-16,-9.));
#16128=CARTESIAN_POINT('Origin',(183.5,0.,-4.6));
#16129=CARTESIAN_POINT('Origin',(210.,2.50000000000003,-9.));
#16130=CARTESIAN_POINT('',(217.,2.50000000000003,-9.));
#16131=CARTESIAN_POINT('Origin',(210.,2.50000000000003,-9.));
#16132=CARTESIAN_POINT('',(217.,2.50000000000003,-8.));
#16133=CARTESIAN_POINT('',(217.,2.50000000000003,-9.));
#16134=CARTESIAN_POINT('Origin',(210.,2.50000000000003,-8.));
#16135=CARTESIAN_POINT('Origin',(210.,2.50000000000003,-8.));
#16136=CARTESIAN_POINT('',(220.,2.50000000000003,-8.));
#16137=CARTESIAN_POINT('Origin',(210.,2.50000000000003,-8.));
#16138=CARTESIAN_POINT('',(220.,2.50000000000003,-7.));
#16139=CARTESIAN_POINT('',(220.,2.50000000000003,-8.));
#16140=CARTESIAN_POINT('Origin',(210.,2.50000000000003,-7.));
#16141=CARTESIAN_POINT('Origin',(210.,2.50000000000003,-7.));
#16142=CARTESIAN_POINT('',(221.1,2.50000000000003,-7.));
#16143=CARTESIAN_POINT('Origin',(210.,2.50000000000003,-7.));
#16144=CARTESIAN_POINT('',(221.1,2.50000000000003,0.));
#16145=CARTESIAN_POINT('',(221.1,2.50000000000003,-7.));
#16146=CARTESIAN_POINT('Origin',(210.,2.50000000000003,0.));
#16147=CARTESIAN_POINT('Origin',(160.,-15.,-3.));
#16148=CARTESIAN_POINT('',(160.,3.94999999999999,-3.));
#16149=CARTESIAN_POINT('',(190.,3.94999999999999,-3.));
#16150=CARTESIAN_POINT('',(190.,3.95,-3.));
#16151=CARTESIAN_POINT('',(190.,15.,-3.));
#16152=CARTESIAN_POINT('',(190.,-15.,-3.));
#16153=CARTESIAN_POINT('',(162.,15.,-3.));
#16154=CARTESIAN_POINT('',(160.,15.,-3.));
#16155=CARTESIAN_POINT('',(160.,13.,-3.));
#16156=CARTESIAN_POINT('Origin',(162.,13.,-3.));
#16157=CARTESIAN_POINT('',(160.,-15.,-3.));
#16158=CARTESIAN_POINT('Origin',(160.,-15.,-3.));
#16159=CARTESIAN_POINT('',(190.,-3.95,-3.));
#16160=CARTESIAN_POINT('',(160.,-3.95,-3.));
#16161=CARTESIAN_POINT('',(190.,-3.95,-3.));
#16162=CARTESIAN_POINT('',(160.,-13.,-3.));
#16163=CARTESIAN_POINT('',(160.,-15.,-3.));
#16164=CARTESIAN_POINT('',(162.,-15.,-3.));
#16165=CARTESIAN_POINT('Origin',(162.,-13.,-3.));
#16166=CARTESIAN_POINT('',(190.,-15.,-3.));
#16167=CARTESIAN_POINT('',(160.,-15.,-3.));
#16168=CARTESIAN_POINT('',(190.,-15.,-3.));
#16169=CARTESIAN_POINT('Origin',(190.,-15.,0.));
#16170=CARTESIAN_POINT('',(190.,3.95,-1.));
#16171=CARTESIAN_POINT('',(190.,3.95,-1.));
#16172=CARTESIAN_POINT('',(190.,-3.95,-1.));
#16173=CARTESIAN_POINT('',(190.,-3.95,-1.));
#16174=CARTESIAN_POINT('',(190.,-3.95,-1.));
#16175=CARTESIAN_POINT('',(190.,-15.,0.));
#16176=CARTESIAN_POINT('',(190.,-15.,0.));
#16177=CARTESIAN_POINT('',(190.,15.,0.));
#16178=CARTESIAN_POINT('',(190.,-15.,0.));
#16179=CARTESIAN_POINT('',(190.,15.,0.));
#16180=CARTESIAN_POINT('Origin',(13.1197502427733,-56.2532019429921,-9.));
#16181=CARTESIAN_POINT('',(212.839139451054,-9.67330222977594,0.));
#16182=CARTESIAN_POINT('',(13.1197502427733,-56.2532019429921,0.));
#16183=CARTESIAN_POINT('',(190.,-15.,-9.));
#16184=CARTESIAN_POINT('',(190.,-15.,-9.));
#16185=CARTESIAN_POINT('',(212.839139451054,-9.67330222977594,-9.));
#16186=CARTESIAN_POINT('',(13.1197502427733,-56.2532019429921,-9.));
#16187=CARTESIAN_POINT('',(212.839139451054,-9.67330222977594,-9.));
#16188=CARTESIAN_POINT('Origin',(210.,2.50000000000003,-9.));
#16189=CARTESIAN_POINT('',(210.,15.,0.));
#16190=CARTESIAN_POINT('Origin',(210.,2.50000000000003,0.));
#16191=CARTESIAN_POINT('',(210.,15.,-9.));
#16192=CARTESIAN_POINT('Origin',(210.,2.50000000000003,-9.));
#16193=CARTESIAN_POINT('',(210.,15.,-9.));
#16194=CARTESIAN_POINT('Origin',(0.,15.,-9.));
#16195=CARTESIAN_POINT('',(0.,15.,0.));
#16196=CARTESIAN_POINT('',(162.,15.,-9.));
#16197=CARTESIAN_POINT('',(0.,15.,-9.));
#16198=CARTESIAN_POINT('',(162.,15.,-9.));
#16199=CARTESIAN_POINT('Origin',(160.,0.,-9.));
#16200=CARTESIAN_POINT('',(160.,13.,-9.));
#16201=CARTESIAN_POINT('',(160.,13.,0.));
#16202=CARTESIAN_POINT('',(160.,7.49999999999998,-9.));
#16203=CARTESIAN_POINT('',(160.,0.,-9.));
#16204=CARTESIAN_POINT('',(160.,7.49999999999997,-15.));
#16205=CARTESIAN_POINT('',(160.,7.49999999999997,-19.));
#16206=CARTESIAN_POINT('',(160.,3.49999999999997,-19.));
#16207=CARTESIAN_POINT('Origin',(160.,3.49999999999997,-15.));
#16208=CARTESIAN_POINT('',(160.,-3.50000000000003,-19.));
#16209=CARTESIAN_POINT('',(160.,-7.50000000000003,-19.));
#16210=CARTESIAN_POINT('',(160.,-7.50000000000003,-15.));
#16211=CARTESIAN_POINT('Origin',(160.,-3.50000000000003,-15.));
#16212=CARTESIAN_POINT('',(160.,-7.50000000000002,-9.));
#16213=CARTESIAN_POINT('',(160.,-7.50000000000003,-19.));
#16214=CARTESIAN_POINT('',(160.,-13.,-9.));
#16215=CARTESIAN_POINT('',(160.,0.,-9.));
#16216=CARTESIAN_POINT('',(160.,-13.,-9.));
#16217=CARTESIAN_POINT('',(160.,-3.95,-1.));
#16218=CARTESIAN_POINT('',(160.,-3.95,-1.));
#16219=CARTESIAN_POINT('',(160.,3.95,-1.));
#16220=CARTESIAN_POINT('',(160.,-3.95,-1.));
#16221=CARTESIAN_POINT('',(160.,3.95,-1.));
#16222=CARTESIAN_POINT('Origin',(1.73472347597681E-15,-15.,-9.));
#16223=CARTESIAN_POINT('',(162.,-15.,-9.));
#16224=CARTESIAN_POINT('',(162.,-15.,-9.));
#16225=CARTESIAN_POINT('',(1.73472347597681E-15,-15.,-9.));
#16226=CARTESIAN_POINT('Origin',(0.,0.,-9.));
#16227=CARTESIAN_POINT('',(169.886751345948,7.49999999999998,-9.));
#16228=CARTESIAN_POINT('',(167.,7.49999999999998,-9.));
#16229=CARTESIAN_POINT('Origin',(162.,13.,-9.));
#16230=CARTESIAN_POINT('Origin',(162.,-13.,-9.));
#16231=CARTESIAN_POINT('',(169.886751345948,-7.50000000000002,-9.));
#16232=CARTESIAN_POINT('',(167.,-7.50000000000002,-9.));
#16233=CARTESIAN_POINT('',(169.886751345948,0.,-9.));
#16234=CARTESIAN_POINT('',(169.886751345948,0.,-9.));
#16235=CARTESIAN_POINT('Origin',(0.,0.,0.));
#16236=CARTESIAN_POINT('Origin',(210.,2.50000000000003,-7.));
#16237=CARTESIAN_POINT('Origin',(210.,2.50000000000003,-8.));
#16238=CARTESIAN_POINT('Origin',(162.,-13.,-9.));
#16239=CARTESIAN_POINT('Origin',(162.,13.,-9.));
#16240=CARTESIAN_POINT('Origin',(185.75,0.,-4.6));
#16241=CARTESIAN_POINT('Origin',(173.75,0.,-4.6));
#16242=CARTESIAN_POINT('Origin',(167.,-7.50000000000002,-19.));
#16243=CARTESIAN_POINT('',(167.,-7.50000000000002,-15.));
#16244=CARTESIAN_POINT('',(167.,-7.50000000000002,-14.));
#16245=CARTESIAN_POINT('',(167.,-7.50000000000002,-19.));
#16246=CARTESIAN_POINT('',(164.834936490539,-7.50000000000002,-17.75));
#16247=CARTESIAN_POINT('',(160.,-7.50000000000003,-15.));
#16248=CARTESIAN_POINT('Origin',(167.,-7.50000000000002,-19.));
#16249=CARTESIAN_POINT('',(167.,-3.50000000000002,-19.));
#16250=CARTESIAN_POINT('Origin',(167.,-3.50000000000002,-15.));
#16251=CARTESIAN_POINT('',(167.,3.49999999999998,-19.));
#16252=CARTESIAN_POINT('',(167.,-7.50000000000002,-19.));
#16253=CARTESIAN_POINT('',(167.,7.49999999999998,-15.));
#16254=CARTESIAN_POINT('Origin',(167.,3.49999999999998,-15.));
#16255=CARTESIAN_POINT('',(167.,7.49999999999998,-14.));
#16256=CARTESIAN_POINT('',(167.,7.49999999999998,-19.));
#16257=CARTESIAN_POINT('',(167.,-7.50000000000002,-14.));
#16258=CARTESIAN_POINT('Origin',(167.,7.49999999999998,-19.));
#16259=CARTESIAN_POINT('',(164.834936490539,7.49999999999998,-17.75));
#16260=CARTESIAN_POINT('',(167.,7.49999999999998,-15.));
#16261=CARTESIAN_POINT('Origin',(0.,0.,-19.));
#16262=CARTESIAN_POINT('',(167.,-3.50000000000002,-19.));
#16263=CARTESIAN_POINT('',(160.,3.49999999999997,-19.));
#16264=CARTESIAN_POINT('Origin',(-4.33680868994196E-16,3.49999999999995,
-15.));
#16265=CARTESIAN_POINT('Origin',(4.33680868994207E-16,-3.50000000000005,
-15.));
#16266=CARTESIAN_POINT('Origin',(167.,-7.50000000000002,-14.));
#16267=CARTESIAN_POINT('Origin',(0.,0.,-1.));
#16268=CARTESIAN_POINT('',(190.,-3.95,-1.));
#16269=CARTESIAN_POINT('',(190.,3.95,-1.));
#16270=CARTESIAN_POINT('Origin',(190.,3.95,-1.));
#16271=CARTESIAN_POINT('Origin',(190.,-3.95,-1.));
#18835=UNCERTAINTY_MEASURE_WITH_UNIT(LENGTH_MEASURE(0.01),#18868,
'DISTANCE_ACCURACY_VALUE',
'Maximum model space distance between geometric entities at asserted c
onnectivities');
#18849=UNCERTAINTY_MEASURE_WITH_UNIT(LENGTH_MEASURE(0.01),#18868,
'DISTANCE_ACCURACY_VALUE',
'Maximum model space distance between geometric entities at asserted c
onnectivities');
#18853=(
GEOMETRIC_REPRESENTATION_CONTEXT(3)
GLOBAL_UNCERTAINTY_ASSIGNED_CONTEXT((#18835))
GLOBAL_UNIT_ASSIGNED_CONTEXT((#18868,#18870,#18871))
REPRESENTATION_CONTEXT('','3D')
);
#18867=(
GEOMETRIC_REPRESENTATION_CONTEXT(3)
GLOBAL_UNCERTAINTY_ASSIGNED_CONTEXT((#18849))
GLOBAL_UNIT_ASSIGNED_CONTEXT((#18868,#18870,#18871))
REPRESENTATION_CONTEXT('','3D')
);
#18868=(
LENGTH_UNIT()
NAMED_UNIT(*)
SI_UNIT(.MILLI.,.METRE.)
);
#18870=(
NAMED_UNIT(*)
PLANE_ANGLE_UNIT()
SI_UNIT($,.RADIAN.)
);
#18871=(
NAMED_UNIT(*)
SI_UNIT($,.STERADIAN.)
SOLID_ANGLE_UNIT()
);
#18875=SHAPE_DEFINITION_REPRESENTATION(#18892,#18937);
#18892=PRODUCT_DEFINITION_SHAPE('',$,#18955);
#18937=SHAPE_REPRESENTATION('',(#11306),#18853);
#18951=PRODUCT_DEFINITION_CONTEXT('part definition',#19004,'design');
#18955=PRODUCT_DEFINITION('Idler End Bracket 1','Idler End Bracket 1',#18972,
#18951);
#18972=PRODUCT_DEFINITION_FORMATION('',$,#19009);
#19004=APPLICATION_CONTEXT(
'Core Data for Automotive Mechanical Design Process');
#19005=PRODUCT_CONTEXT('part definition',#19004,'mechanical');
#19009=PRODUCT('Idler End Bracket 1','Idler End Bracket 1',$,(#19005));
#19024=PRESENTATION_STYLE_ASSIGNMENT((#19030));
#19030=SURFACE_STYLE_USAGE(.BOTH.,#19036);
#19036=SURFACE_SIDE_STYLE('',(#19042));
#19042=SURFACE_STYLE_FILL_AREA(#19048);
#19048=FILL_AREA_STYLE('Opaque(20,51,87)',(#19054));
#19054=FILL_AREA_STYLE_COLOUR('Opaque(20,51,87)',#19060);
#19060=COLOUR_RGB('Opaque(20,51,87)',0.0784313725490196,0.2,0.341176470588235);
ENDSEC;
END-ISO-10303-21;
